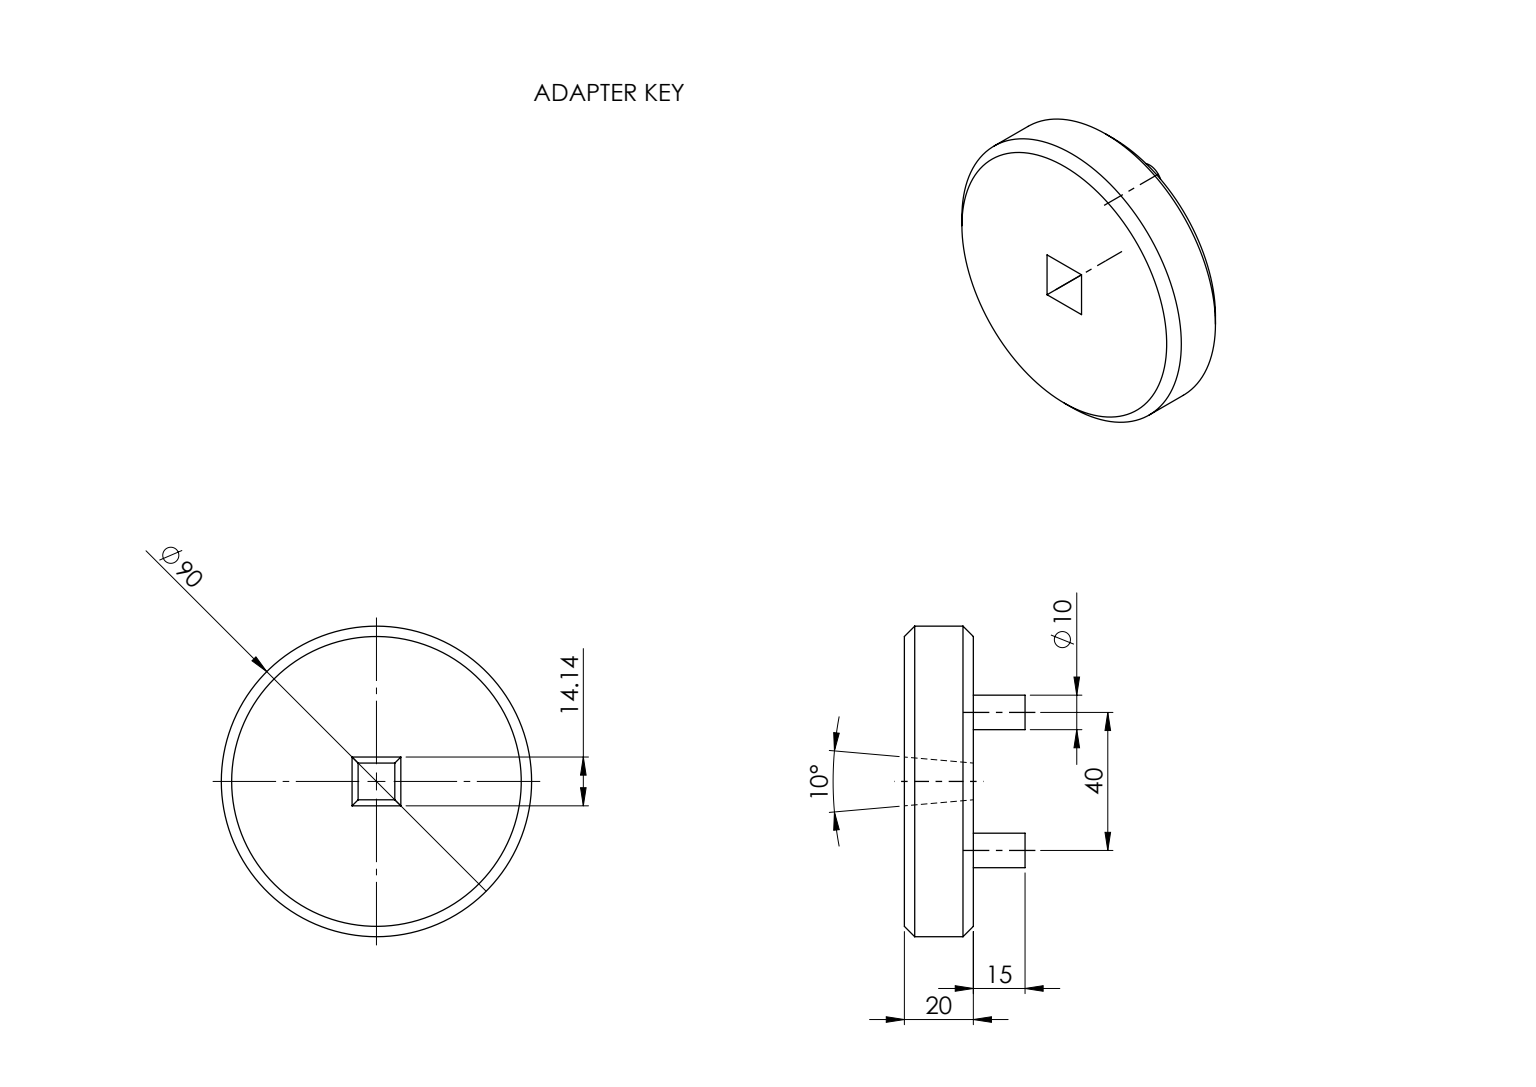
ISO-10303-21;
HEADER;
FILE_DESCRIPTION (('STEP AP203'),
    '1' );
FILE_NAME ('adapter key.step',
    '2026-09-28T05:57:06',
    ( '' ),
    ( '' ),
    'SwSTEP 2.0',
    'SolidWorks 2026',
    '' );
FILE_SCHEMA (( 'AUTOMOTIVE_DESIGN' ));
ENDSEC;

DATA;
#1=ORIENTED_EDGE ( 'NONE', *, *, #11918, .T. ) ;
#11=AXIS2_PLACEMENT_3D ( 'NONE', #22333, #25786, #11966 ) ;
#126=FACE_OUTER_BOUND ( 'NONE', #13645, .T. ) ;
#159=DIRECTION ( 'NONE',  ( -1.000000000000000000, 0.000000000000000000, 0.000000000000000000 ) ) ;
#483=ORIENTED_EDGE ( 'NONE', *, *, #39890, .F. ) ;
#526=CARTESIAN_POINT ( 'NONE',  ( 0.000000000000000000, 5.321294541346989426, -219.9999999999999716 ) ) ;
#674=CARTESIAN_POINT ( 'NONE',  ( 6.964452268037472749, 6.964452268037473637, -201.2186212422413689 ) ) ;
#785=DIRECTION ( 'NONE',  ( -0.000000000000000000, -0.000000000000000000, 1.000000000000000000 ) ) ;
#953=CARTESIAN_POINT ( 'NONE',  ( -5.000000000000002665, 20.00000000000000000, -235.0000000000000000 ) ) ;
#967=CARTESIAN_POINT ( 'NONE',  ( -2.275517850991317657E-15, -20.00000000000000000, -235.0000000000000000 ) ) ;
#1100=VECTOR ( 'NONE', #32490, 1000.000000000000000 ) ;
#1141=ORIENTED_EDGE ( 'NONE', *, *, #16442, .T. ) ;
#1157=CARTESIAN_POINT ( 'NONE',  ( -45.00000000000000711, 0.000000000000000000, -203.0000000000000000 ) ) ;
#1331=DIRECTION ( 'NONE',  ( 0.000000000000000000, 0.000000000000000000, -1.000000000000000000 ) ) ;
#1487=MANIFOLD_SOLID_BREP ( 'Cavity1', #17003 ) ;
#1498=PRODUCT ( 'adapter key', 'adapter key', '', ( #33542 ) ) ;
#1541=EDGE_LOOP ( 'NONE', ( #15994, #2474, #42330, #20143 ) ) ;
#1544=AXIS2_PLACEMENT_3D ( 'NONE', #42021, #38801, #12243 ) ;
#1593=ORIENTED_EDGE ( 'NONE', *, *, #39837, .F. ) ;
#1636=CARTESIAN_POINT ( 'NONE',  ( -45.00000000000000711, 0.000000000000000000, -217.0000000000000853 ) ) ;
#1647=CARTESIAN_POINT ( 'NONE',  ( 5.000000000000000000, -20.00000000000000000, -235.0000000000000000 ) ) ;
#1763=AXIS2_PLACEMENT_3D ( 'NONE', #7556, #33682, #13996 ) ;
#2026=ADVANCED_FACE ( 'NONE', ( #8164 ), #10577, .F. ) ;
#2078=CARTESIAN_POINT ( 'NONE',  ( 0.000000000000000000, 0.000000000000000000, -200.0000000000000000 ) ) ;
#2080=VECTOR ( 'NONE', #35351, 1000.000000000000000 ) ;
#2296=DIRECTION ( 'NONE',  ( 0.000000000000000000, 0.000000000000000000, -1.000000000000000000 ) ) ;
#2379=DIRECTION ( 'NONE',  ( 0.000000000000000000, 0.000000000000000000, -1.000000000000000000 ) ) ;
#2410=CARTESIAN_POINT ( 'NONE',  ( 0.000000000000000000, 0.000000000000000000, -200.0000000000000000 ) ) ;
#2474=ORIENTED_EDGE ( 'NONE', *, *, #18806, .T. ) ;
#2480=EDGE_CURVE ( 'NONE', #35035, #8964, #11432, .T. ) ;
#2552=CARTESIAN_POINT ( 'NONE',  ( 42.00000000000004974, 0.000000000000000000, -219.9999999999999716 ) ) ;
#2589=FACE_OUTER_BOUND ( 'NONE', #11013, .T. ) ;
#2598=DIRECTION ( 'NONE',  ( 0.08682659386424779191, -0.08682659386424779191, 0.9924325091389669673 ) ) ;
#2602=ORIENTED_EDGE ( 'NONE', *, *, #11918, .F. ) ;
#2615=CARTESIAN_POINT ( 'NONE',  ( -7.071067811865477282, 7.071067811865471064, -200.0000000000000000 ) ) ;
#2639=DIRECTION ( 'NONE',  ( 0.000000000000000000, 0.000000000000000000, -1.000000000000000000 ) ) ;
#2651=EDGE_LOOP ( 'NONE', ( #20661, #18080, #34460, #33121 ) ) ;
#2652=EDGE_LOOP ( 'NONE', ( #37130, #21052, #35179, #1 ) ) ;
#2679=ORIENTED_EDGE ( 'NONE', *, *, #40709, .F. ) ;
#2703=DIRECTION ( 'NONE',  ( 0.000000000000000000, 0.000000000000000000, -1.000000000000000000 ) ) ;
#2844=FACE_OUTER_BOUND ( 'NONE', #29189, .T. ) ;
#2864=ADVANCED_FACE ( 'NONE', ( #37885 ), #20831, .F. ) ;
#2943=AXIS2_PLACEMENT_3D ( 'NONE', #28917, #28711, #6033 ) ;
#3110=AXIS2_PLACEMENT_3D ( 'NONE', #25408, #5334, #8580 ) ;
#3136=VECTOR ( 'NONE', #7346, 1000.000000000000114 ) ;
#3175=CARTESIAN_POINT ( 'NONE',  ( -2.275517850991317657E-15, -20.00000000000000000, -219.9999999999999716 ) ) ;
#3290=DIRECTION ( 'NONE',  ( -0.000000000000000000, -0.000000000000000000, 1.000000000000000000 ) ) ;
#3542=VERTEX_POINT ( 'NONE', #1157 ) ;
#3598=DIRECTION ( 'NONE',  ( -0.7071067811865483499, 8.659560562354942719E-17, 0.7071067811865466846 ) ) ;
#3686=CARTESIAN_POINT ( 'NONE',  ( 5.000000000000000000, -20.00000000000000000, -219.9999999999999716 ) ) ;
#3707=ADVANCED_FACE ( 'NONE', ( #31585 ), #42117, .F. ) ;
#3843=DIRECTION ( 'NONE',  ( 0.000000000000000000, 0.000000000000000000, -1.000000000000000000 ) ) ;
#4412=FACE_OUTER_BOUND ( 'NONE', #14165, .T. ) ;
#4607=CARTESIAN_POINT ( 'NONE',  ( -5.321294541346989426, -5.321294541346989426, -219.9999999999999716 ) ) ;
#4626=DIRECTION ( 'NONE',  ( -1.000000000000000000, 0.000000000000000000, 0.000000000000000000 ) ) ;
#4650=CARTESIAN_POINT ( 'NONE',  ( 7.071067811865472841, 7.071067811865472841, -200.0000000000000000 ) ) ;
#4654=CARTESIAN_POINT ( 'NONE',  ( -7.071067811865477282, -7.071067811865472841, -200.0000000000000000 ) ) ;
#4922=DIRECTION ( 'NONE',  ( 0.000000000000000000, -0.9961946980917455452, -0.08715574274765837404 ) ) ;
#5010=AXIS2_PLACEMENT_3D ( 'NONE', #18603, #2639, #41891 ) ;
#5035=DIRECTION ( 'NONE',  ( -0.9961946980917455452, 0.000000000000000000, -0.08715574274765837404 ) ) ;
#5279=ORIENTED_EDGE ( 'NONE', *, *, #9308, .F. ) ;
#5319=CARTESIAN_POINT ( 'NONE',  ( 0.000000000000000000, 0.000000000000000000, -219.9999999999999716 ) ) ;
#5334=DIRECTION ( 'NONE',  ( 0.000000000000000000, 0.000000000000000000, -1.000000000000000000 ) ) ;
#5395=ORIENTED_EDGE ( 'NONE', *, *, #30592, .T. ) ;
#5451=PLANE ( 'NONE',  #28654 ) ;
#5465=ORIENTED_EDGE ( 'NONE', *, *, #12760, .F. ) ;
#5647=CARTESIAN_POINT ( 'NONE',  ( 0.000000000000000000, 20.00000000000000000, -235.0000000000000000 ) ) ;
#5755=ORIENTED_EDGE ( 'NONE', *, *, #38350, .F. ) ;
#5887=ORIENTED_EDGE ( 'NONE', *, *, #16876, .F. ) ;
#5935=AXIS2_PLACEMENT_3D ( 'NONE', #14018, #2703, #6942 ) ;
#5940=( NAMED_UNIT ( * ) PLANE_ANGLE_UNIT ( ) SI_UNIT ( $, .RADIAN. ) );
#6033=DIRECTION ( 'NONE',  ( -1.000000000000000000, 0.000000000000000000, 0.000000000000000000 ) ) ;
#6444=CARTESIAN_POINT ( 'NONE',  ( 0.000000000000000000, 0.000000000000000000, -219.9999999999999716 ) ) ;
#6566=AXIS2_PLACEMENT_3D ( 'NONE', #10357, #39929, #7353 ) ;
#6633=DIRECTION ( 'NONE',  ( 1.000000000000000000, -0.000000000000000000, -0.000000000000000000 ) ) ;
#6797=VECTOR ( 'NONE', #10559, 1000.000000000000000 ) ;
#6839=FACE_OUTER_BOUND ( 'NONE', #22128, .T. ) ;
#6843=CIRCLE ( 'NONE', #42657, 5.000000000000002665 ) ;
#6856=DIRECTION ( 'NONE',  ( -1.000000000000000000, 0.000000000000000000, -0.000000000000000000 ) ) ;
#6863=EDGE_CURVE ( 'NONE', #25211, #17989, #19820, .T. ) ;
#6942=DIRECTION ( 'NONE',  ( -1.000000000000000000, 0.000000000000000000, 0.000000000000000000 ) ) ;
#6947=CARTESIAN_POINT ( 'NONE',  ( -2.275517850991317657E-15, -20.00000000000000000, -235.0000000000000000 ) ) ;
#6976=EDGE_CURVE ( 'NONE', #21643, #18815, #29301, .T. ) ;
#6984=LINE ( 'NONE', #526, #42165 ) ;
#7000=AXIS2_PLACEMENT_3D ( 'NONE', #27316, #785, #27529 ) ;
#7012=DIRECTION ( 'NONE',  ( -1.000000000000000000, 0.000000000000000000, -0.000000000000000000 ) ) ;
#7136=FACE_BOUND ( 'NONE', #35464, .T. ) ;
#7294=CARTESIAN_POINT ( 'NONE',  ( 7.071067811865477282, -7.071067811865471064, -200.0000000000000000 ) ) ;
#7346=DIRECTION ( 'NONE',  ( 0.08682659386424779191, 0.08682659386424779191, 0.9924325091389669673 ) ) ;
#7353=DIRECTION ( 'NONE',  ( -1.000000000000000000, 0.000000000000000000, -0.000000000000000000 ) ) ;
#7454=EDGE_CURVE ( 'NONE', #27111, #16738, #32754, .T. ) ;
#7556=CARTESIAN_POINT ( 'NONE',  ( -2.275517850991317657E-15, -20.00000000000000000, -235.0000000000000000 ) ) ;
#7576=CIRCLE ( 'NONE', #11, 5.000000000000002665 ) ;
#7595=DIRECTION ( 'NONE',  ( 0.9961946980917455452, 0.000000000000000000, -0.08715574274765837404 ) ) ;
#7679=DIRECTION ( 'NONE',  ( 0.000000000000000000, 0.9961946980917455452, -0.08715574274765837404 ) ) ;
#7755=EDGE_CURVE ( 'NONE', #14989, #27111, #11989, .T. ) ;
#7817=FACE_OUTER_BOUND ( 'NONE', #27002, .T. ) ;
#8134=DIRECTION ( 'NONE',  ( 0.000000000000000000, 0.000000000000000000, 1.000000000000000000 ) ) ;
#8164=FACE_OUTER_BOUND ( 'NONE', #20948, .T. ) ;
#8171=DIRECTION ( 'NONE',  ( 1.000000000000000000, 0.000000000000000000, 0.000000000000000000 ) ) ;
#8303=PRODUCT_DEFINITION ( 'UNKNOWN', '', #24948, #36055 ) ;
#8326=LINE ( 'NONE', #21042, #9603 ) ;
#8516=ORIENTED_EDGE ( 'NONE', *, *, #38069, .F. ) ;
#8544=ORIENTED_EDGE ( 'NONE', *, *, #12979, .T. ) ;
#8580=DIRECTION ( 'NONE',  ( -1.000000000000000000, 0.000000000000000000, 0.000000000000000000 ) ) ;
#8659=ORIENTED_EDGE ( 'NONE', *, *, #39837, .T. ) ;
#8684=CIRCLE ( 'NONE', #26592, 45.00000000000000711 ) ;
#8737=ORIENTED_EDGE ( 'NONE', *, *, #22756, .T. ) ;
#8756=CARTESIAN_POINT ( 'NONE',  ( 0.000000000000000000, 0.000000000000000000, -217.0000000000000853 ) ) ;
#8860=ORIENTED_EDGE ( 'NONE', *, *, #30592, .F. ) ;
#8964=VERTEX_POINT ( 'NONE', #34365 ) ;
#9066=ADVANCED_FACE ( 'NONE', ( #7817 ), #30906, .F. ) ;
#9301=EDGE_CURVE ( 'NONE', #13682, #12005, #6843, .T. ) ;
#9308=EDGE_CURVE ( 'NONE', #32599, #21643, #15789, .T. ) ;
#9399=DIRECTION ( 'NONE',  ( 0.000000000000000000, 0.000000000000000000, 1.000000000000000000 ) ) ;
#9603=VECTOR ( 'NONE', #11321, 1000.000000000000000 ) ;
#9635=CYLINDRICAL_SURFACE ( 'NONE', #7000, 5.000000000000002665 ) ;
#9644=EDGE_LOOP ( 'NONE', ( #21891, #30300, #22496, #15785 ) ) ;
#10152=FACE_OUTER_BOUND ( 'NONE', #39088, .T. ) ;
#10209=ORIENTED_EDGE ( 'NONE', *, *, #38350, .T. ) ;
#10271=ORIENTED_EDGE ( 'NONE', *, *, #41214, .F. ) ;
#10357=CARTESIAN_POINT ( 'NONE',  ( 0.000000000000000000, 0.000000000000000000, -219.9999999999999716 ) ) ;
#10378=ADVANCED_FACE ( 'NONE', ( #34632, #27507 ), #13521, .F. ) ;
#10417=CARTESIAN_POINT ( 'NONE',  ( 7.071067811865472841, -7.071067811865472841, -200.0000000000000000 ) ) ;
#10540=CARTESIAN_POINT ( 'NONE',  ( 5.000000000000002665, 20.00000000000000000, -219.9999999999999716 ) ) ;
#10559=DIRECTION ( 'NONE',  ( -0.000000000000000000, -0.000000000000000000, 1.000000000000000000 ) ) ;
#10577=PLANE ( 'NONE',  #12775 ) ;
#10589=DIRECTION ( 'NONE',  ( -1.000000000000000000, 0.000000000000000000, 0.000000000000000000 ) ) ;
#10590=ADVANCED_FACE ( 'NONE', ( #4412 ), #22716, .T. ) ;
#10848=AXIS2_PLACEMENT_3D ( 'NONE', #6947, #1331, #10589 ) ;
#10918=DIRECTION ( 'NONE',  ( -0.000000000000000000, -1.000000000000000000, -0.000000000000000000 ) ) ;
#11013=EDGE_LOOP ( 'NONE', ( #11087, #37618, #18353, #1593 ) ) ;
#11087=ORIENTED_EDGE ( 'NONE', *, *, #23326, .F. ) ;
#11112=DIRECTION ( 'NONE',  ( 0.000000000000000000, 0.000000000000000000, 1.000000000000000000 ) ) ;
#11133=LINE ( 'NONE', #18253, #42479 ) ;
#11321=DIRECTION ( 'NONE',  ( -1.000000000000000000, 0.000000000000000000, 0.000000000000000000 ) ) ;
#11331=ORIENTED_EDGE ( 'NONE', *, *, #20682, .F. ) ;
#11377=CIRCLE ( 'NONE', #1763, 5.000000000000002665 ) ;
#11382=CARTESIAN_POINT ( 'NONE',  ( -2.275517850991317657E-15, -20.00000000000000000, -235.0000000000000000 ) ) ;
#11432=CIRCLE ( 'NONE', #12117, 5.000000000000002665 ) ;
#11492=DIRECTION ( 'NONE',  ( -0.08682659386424779191, -0.08682659386424779191, 0.9924325091389669673 ) ) ;
#11559=AXIS2_PLACEMENT_3D ( 'NONE', #40001, #42386, #22553 ) ;
#11596=ORIENTED_EDGE ( 'NONE', *, *, #2480, .F. ) ;
#11632=CARTESIAN_POINT ( 'NONE',  ( -45.00000000000000711, 0.000000000000000000, -200.0000000000000000 ) ) ;
#11721=VECTOR ( 'NONE', #18934, 1000.000000000000114 ) ;
#11857=APPLICATION_CONTEXT ( 'configuration controlled 3d designs of mechanical parts and assemblies' ) ;
#11870=EDGE_CURVE ( 'NONE', #17989, #25211, #11377, .T. ) ;
#11918=EDGE_CURVE ( 'NONE', #28029, #16738, #39924, .T. ) ;
#11966=DIRECTION ( 'NONE',  ( -1.000000000000000000, 0.000000000000000000, 0.000000000000000000 ) ) ;
#11989=LINE ( 'NONE', #38534, #22609 ) ;
#11992=FACE_OUTER_BOUND ( 'NONE', #35700, .T. ) ;
#12005=VERTEX_POINT ( 'NONE', #15500 ) ;
#12066=CARTESIAN_POINT ( 'NONE',  ( 45.00000000000000711, 5.510910596163090344E-15, -203.0000000000000000 ) ) ;
#12076=ORIENTED_EDGE ( 'NONE', *, *, #9301, .F. ) ;
#12117=AXIS2_PLACEMENT_3D ( 'NONE', #3175, #13911, #159 ) ;
#12133=EDGE_LOOP ( 'NONE', ( #33495, #8860, #16467, #13801 ) ) ;
#12243=DIRECTION ( 'NONE',  ( -1.000000000000000000, 0.000000000000000000, 0.000000000000000000 ) ) ;
#12301=VECTOR ( 'NONE', #30444, 1000.000000000000000 ) ;
#12357=CARTESIAN_POINT ( 'NONE',  ( 0.000000000000000000, 0.000000000000000000, -200.0000000000000000 ) ) ;
#12505=CARTESIAN_POINT ( 'NONE',  ( 0.000000000000000000, 0.000000000000000000, -219.9999999999999716 ) ) ;
#12537=DIRECTION ( 'NONE',  ( -1.000000000000000000, 0.000000000000000000, -0.000000000000000000 ) ) ;
#12651=VERTEX_POINT ( 'NONE', #7294 ) ;
#12747=AXIS2_PLACEMENT_3D ( 'NONE', #41976, #9399, #35532 ) ;
#12760=EDGE_CURVE ( 'NONE', #23937, #42482, #35502, .T. ) ;
#12775=AXIS2_PLACEMENT_3D ( 'NONE', #24574, #4922, #37722 ) ;
#12979=EDGE_CURVE ( 'NONE', #16950, #13797, #16502, .T. ) ;
#13267=DIRECTION ( 'NONE',  ( -1.000000000000000000, -0.000000000000000000, -0.000000000000000000 ) ) ;
#13298=DIRECTION ( 'NONE',  ( -0.000000000000000000, -0.000000000000000000, -1.000000000000000000 ) ) ;
#13521=PLANE ( 'NONE',  #24803 ) ;
#13645=EDGE_LOOP ( 'NONE', ( #17252, #15517 ) ) ;
#13656=FACE_OUTER_BOUND ( 'NONE', #1541, .T. ) ;
#13682=VERTEX_POINT ( 'NONE', #953 ) ;
#13797=VERTEX_POINT ( 'NONE', #4607 ) ;
#13801=ORIENTED_EDGE ( 'NONE', *, *, #7755, .T. ) ;
#13832=( GEOMETRIC_REPRESENTATION_CONTEXT ( 3 ) GLOBAL_UNCERTAINTY_ASSIGNED_CONTEXT ( ( #33340 ) ) GLOBAL_UNIT_ASSIGNED_CONTEXT ( ( #31640, #5940, #25165 ) ) REPRESENTATION_CONTEXT ( 'NONE', 'WORKASPACE' ) );
#13911=DIRECTION ( 'NONE',  ( 0.000000000000000000, 0.000000000000000000, -1.000000000000000000 ) ) ;
#13930=VECTOR ( 'NONE', #2379, 1000.000000000000000 ) ;
#13996=DIRECTION ( 'NONE',  ( -1.000000000000000000, 0.000000000000000000, 0.000000000000000000 ) ) ;
#14018=CARTESIAN_POINT ( 'NONE',  ( 0.000000000000000000, 20.00000000000000000, -219.9999999999999716 ) ) ;
#14158=AXIS2_PLACEMENT_3D ( 'NONE', #31807, #5035, #28979 ) ;
#14165=EDGE_LOOP ( 'NONE', ( #30572, #5279, #8659, #38093 ) ) ;
#14623=ADVANCED_FACE ( 'NONE', ( #38005 ), #35268, .T. ) ;
#14777=DIRECTION ( 'NONE',  ( -0.000000000000000000, -0.000000000000000000, 1.000000000000000000 ) ) ;
#14868=DIRECTION ( 'NONE',  ( 0.000000000000000000, 0.000000000000000000, -1.000000000000000000 ) ) ;
#14989=VERTEX_POINT ( 'NONE', #39478 ) ;
#15381=ADVANCED_FACE ( 'NONE', ( #42426 ), #9635, .T. ) ;
#15500=CARTESIAN_POINT ( 'NONE',  ( 5.000000000000002665, 20.00000000000000000, -235.0000000000000000 ) ) ;
#15517=ORIENTED_EDGE ( 'NONE', *, *, #11870, .T. ) ;
#15528=DIRECTION ( 'NONE',  ( 0.000000000000000000, 0.000000000000000000, 1.000000000000000000 ) ) ;
#15785=ORIENTED_EDGE ( 'NONE', *, *, #2480, .T. ) ;
#15789=CIRCLE ( 'NONE', #33719, 42.00000000000001421 ) ;
#15836=CIRCLE ( 'NONE', #39980, 5.000000000000002665 ) ;
#15858=ORIENTED_EDGE ( 'NONE', *, *, #35195, .T. ) ;
#15994=ORIENTED_EDGE ( 'NONE', *, *, #29097, .T. ) ;
#16130=ORIENTED_EDGE ( 'NONE', *, *, #31655, .F. ) ;
#16145=EDGE_CURVE ( 'NONE', #14989, #28029, #6984, .T. ) ;
#16200=ORIENTED_EDGE ( 'NONE', *, *, #18037, .T. ) ;
#16205=CARTESIAN_POINT ( 'NONE',  ( -2.275517850991317657E-15, -20.00000000000000000, -235.0000000000000000 ) ) ;
#16309=ORIENTED_EDGE ( 'NONE', *, *, #12760, .T. ) ;
#16354=VECTOR ( 'NONE', #11492, 1000.000000000000114 ) ;
#16442=EDGE_CURVE ( 'NONE', #16950, #12651, #39986, .T. ) ;
#16467=ORIENTED_EDGE ( 'NONE', *, *, #22649, .T. ) ;
#16502=LINE ( 'NONE', #32522, #26548 ) ;
#16738=VERTEX_POINT ( 'NONE', #32984 ) ;
#16876=EDGE_CURVE ( 'NONE', #42482, #23937, #26361, .T. ) ;
#16950=VERTEX_POINT ( 'NONE', #21243 ) ;
#16977=DIRECTION ( 'NONE',  ( -1.000000000000000000, 0.000000000000000000, 0.000000000000000000 ) ) ;
#17003=CLOSED_SHELL ( 'NONE', ( #18808, #14623, #29395, #30885, #30210, #10378, #24136, #20403, #42288, #22994, #15381, #23992, #22502, #10590, #3707, #2864, #9066, #2026 ) ) ;
#17162=ORIENTED_EDGE ( 'NONE', *, *, #20682, .T. ) ;
#17252=ORIENTED_EDGE ( 'NONE', *, *, #6863, .T. ) ;
#17551=CARTESIAN_POINT ( 'NONE',  ( 0.000000000000000000, 0.000000000000000000, -203.0000000000000000 ) ) ;
#17817=LINE ( 'NONE', #31440, #32266 ) ;
#17898=APPLICATION_CONTEXT ( 'configuration controlled 3d designs of mechanical parts and assemblies' ) ;
#17989=VERTEX_POINT ( 'NONE', #31791 ) ;
#18025=DIRECTION ( 'NONE',  ( -1.000000000000000000, 0.000000000000000000, 0.000000000000000000 ) ) ;
#18037=EDGE_CURVE ( 'NONE', #8964, #35035, #27055, .T. ) ;
#18080=ORIENTED_EDGE ( 'NONE', *, *, #22649, .F. ) ;
#18187=LINE ( 'NONE', #41048, #16354 ) ;
#18253=CARTESIAN_POINT ( 'NONE',  ( -5.321294541346989426, 0.000000000000000000, -219.9999999999999716 ) ) ;
#18353=ORIENTED_EDGE ( 'NONE', *, *, #29097, .F. ) ;
#18496=ORIENTED_EDGE ( 'NONE', *, *, #11870, .F. ) ;
#18509=EDGE_CURVE ( 'NONE', #3542, #38155, #24192, .T. ) ;
#18603=CARTESIAN_POINT ( 'NONE',  ( -2.275517850991317657E-15, -20.00000000000000000, -219.9999999999999716 ) ) ;
#18667=DIRECTION ( 'NONE',  ( -1.000000000000000000, 0.000000000000000000, 0.000000000000000000 ) ) ;
#18795=DIRECTION ( 'NONE',  ( -1.000000000000000000, 0.000000000000000000, 0.000000000000000000 ) ) ;
#18806=EDGE_CURVE ( 'NONE', #18815, #38638, #22005, .T. ) ;
#18808=ADVANCED_FACE ( 'NONE', ( #2589 ), #31888, .T. ) ;
#18815=VERTEX_POINT ( 'NONE', #12066 ) ;
#18886=EDGE_LOOP ( 'NONE', ( #5465, #36501, #39209, #29608 ) ) ;
#18934=DIRECTION ( 'NONE',  ( -0.7071067811865459074, 0.000000000000000000, -0.7071067811865491270 ) ) ;
#19139=CARTESIAN_POINT ( 'NONE',  ( 0.000000000000000000, 20.00000000000000000, -219.9999999999999716 ) ) ;
#19299=CYLINDRICAL_SURFACE ( 'NONE', #11559, 45.00000000000000711 ) ;
#19340=AXIS2_PLACEMENT_3D ( 'NONE', #11382, #24580, #8171 ) ;
#19343=DIRECTION ( 'NONE',  ( 0.000000000000000000, 0.000000000000000000, -1.000000000000000000 ) ) ;
#19407=AXIS2_PLACEMENT_3D ( 'NONE', #12505, #15528, #38427 ) ;
#19554=LINE ( 'NONE', #38996, #2080 ) ;
#19713=CARTESIAN_POINT ( 'NONE',  ( 45.00000000000000711, 5.510910596163090344E-15, -217.0000000000000853 ) ) ;
#19820=CIRCLE ( 'NONE', #10848, 5.000000000000002665 ) ;
#19946=VECTOR ( 'NONE', #3598, 1000.000000000000000 ) ;
#19992=CYLINDRICAL_SURFACE ( 'NONE', #28417, 5.000000000000002665 ) ;
#20143=ORIENTED_EDGE ( 'NONE', *, *, #18509, .F. ) ;
#20241=ORIENTED_EDGE ( 'NONE', *, *, #20405, .F. ) ;
#20300=EDGE_CURVE ( 'NONE', #38638, #38155, #8684, .T. ) ;
#20403=ADVANCED_FACE ( 'NONE', ( #31645 ), #35518, .T. ) ;
#20405=EDGE_CURVE ( 'NONE', #25211, #35035, #31220, .T. ) ;
#20412=VERTEX_POINT ( 'NONE', #27973 ) ;
#20419=EDGE_CURVE ( 'NONE', #37668, #27111, #41100, .T. ) ;
#20520=VECTOR ( 'NONE', #6633, 1000.000000000000000 ) ;
#20580=DIRECTION ( 'NONE',  ( 0.000000000000000000, 0.000000000000000000, -1.000000000000000000 ) ) ;
#20661=ORIENTED_EDGE ( 'NONE', *, *, #16145, .F. ) ;
#20682=EDGE_CURVE ( 'NONE', #21356, #20412, #24546, .T. ) ;
#20831=PLANE ( 'NONE',  #38306 ) ;
#20887=DIRECTION ( 'NONE',  ( -0.000000000000000000, -0.000000000000000000, 1.000000000000000000 ) ) ;
#20948=EDGE_LOOP ( 'NONE', ( #5755, #38517, #8544, #5395 ) ) ;
#21042=CARTESIAN_POINT ( 'NONE',  ( 7.071067811865472841, -7.071067811865472841, -200.0000000000000000 ) ) ;
#21052=ORIENTED_EDGE ( 'NONE', *, *, #7755, .F. ) ;
#21243=CARTESIAN_POINT ( 'NONE',  ( 5.321294541346989426, -5.321294541346989426, -219.9999999999999716 ) ) ;
#21356=VERTEX_POINT ( 'NONE', #10540 ) ;
#21384=DIRECTION ( 'NONE',  ( 0.7071067811865459074, 8.659560562354911904E-17, -0.7071067811865491270 ) ) ;
#21643=VERTEX_POINT ( 'NONE', #37953 ) ;
#21842=CARTESIAN_POINT ( 'NONE',  ( 0.000000000000000000, 20.00000000000000000, -235.0000000000000000 ) ) ;
#21891=ORIENTED_EDGE ( 'NONE', *, *, #35192, .F. ) ;
#22005=LINE ( 'NONE', #32583, #13930 ) ;
#22096=DIRECTION ( 'NONE',  ( -0.000000000000000000, -0.000000000000000000, 1.000000000000000000 ) ) ;
#22128=EDGE_LOOP ( 'NONE', ( #12076, #38318, #23767, #483 ) ) ;
#22333=CARTESIAN_POINT ( 'NONE',  ( 0.000000000000000000, 20.00000000000000000, -235.0000000000000000 ) ) ;
#22438=AXIS2_PLACEMENT_3D ( 'NONE', #12357, #22096, #23313 ) ;
#22473=AXIS2_PLACEMENT_3D ( 'NONE', #2078, #2296, #18025 ) ;
#22496=ORIENTED_EDGE ( 'NONE', *, *, #20405, .T. ) ;
#22502=ADVANCED_FACE ( 'NONE', ( #11992 ), #41769, .T. ) ;
#22550=CARTESIAN_POINT ( 'NONE',  ( -7.071067811865472841, -7.071067811865472841, -200.0000000000000000 ) ) ;
#22553=DIRECTION ( 'NONE',  ( -1.000000000000000000, 0.000000000000000000, 0.000000000000000000 ) ) ;
#22609=VECTOR ( 'NONE', #38116, 1000.000000000000114 ) ;
#22649=EDGE_CURVE ( 'NONE', #13797, #14989, #11133, .T. ) ;
#22716=CONICAL_SURFACE ( 'NONE', #40617, 45.00000000000000711, 0.7853981633974459475 ) ;
#22756=EDGE_CURVE ( 'NONE', #38155, #38638, #31482, .T. ) ;
#22911=FACE_BOUND ( 'NONE', #28242, .T. ) ;
#22994=ADVANCED_FACE ( 'NONE', ( #126 ), #33770, .T. ) ;
#23138=DIRECTION ( 'NONE',  ( 1.000000000000000000, 0.000000000000000000, 0.000000000000000000 ) ) ;
#23313=DIRECTION ( 'NONE',  ( -1.000000000000000000, 0.000000000000000000, 0.000000000000000000 ) ) ;
#23326=EDGE_CURVE ( 'NONE', #21643, #32599, #29309, .T. ) ;
#23333=FACE_BOUND ( 'NONE', #2651, .T. ) ;
#23352=VECTOR ( 'NONE', #29633, 1000.000000000000000 ) ;
#23615=VECTOR ( 'NONE', #14868, 1000.000000000000000 ) ;
#23680=DIRECTION ( 'NONE',  ( -1.000000000000000000, 0.000000000000000000, 0.000000000000000000 ) ) ;
#23745=LINE ( 'NONE', #36898, #12301 ) ;
#23767=ORIENTED_EDGE ( 'NONE', *, *, #41214, .T. ) ;
#23885=PRODUCT_DEFINITION_SHAPE ( 'NONE', 'NONE',  #8303 ) ;
#23894=AXIS2_PLACEMENT_3D ( 'NONE', #5319, #8134, #34686 ) ;
#23937=VERTEX_POINT ( 'NONE', #41889 ) ;
#23992=ADVANCED_FACE ( 'NONE', ( #2844 ), #5451, .T. ) ;
#24093=ORIENTED_EDGE ( 'NONE', *, *, #18806, .F. ) ;
#24136=ADVANCED_FACE ( 'NONE', ( #10152, #7136, #22911, #23333 ), #36907, .T. ) ;
#24189=ORIENTED_EDGE ( 'NONE', *, *, #35192, .T. ) ;
#24192=LINE ( 'NONE', #11632, #23615 ) ;
#24335=DIRECTION ( 'NONE',  ( -0.000000000000000000, 1.000000000000000000, -0.000000000000000000 ) ) ;
#24426=ORIENTED_EDGE ( 'NONE', *, *, #9308, .T. ) ;
#24546=CIRCLE ( 'NONE', #5935, 5.000000000000002665 ) ;
#24574=CARTESIAN_POINT ( 'NONE',  ( 7.071067811865472841, -7.071067811865472841, -200.0000000000000000 ) ) ;
#24580=DIRECTION ( 'NONE',  ( -0.000000000000000000, -0.000000000000000000, 1.000000000000000000 ) ) ;
#24743=CARTESIAN_POINT ( 'NONE',  ( 0.000000000000000000, 0.000000000000000000, 0.000000000000000000 ) ) ;
#24803=AXIS2_PLACEMENT_3D ( 'NONE', #37205, #37429, #6856 ) ;
#24948=PRODUCT_DEFINITION_FORMATION_WITH_SPECIFIED_SOURCE ( 'ANY', '', #1498, .NOT_KNOWN. ) ;
#25165=( NAMED_UNIT ( * ) SI_UNIT ( $, .STERADIAN. ) SOLID_ANGLE_UNIT ( ) );
#25211=VERTEX_POINT ( 'NONE', #41304 ) ;
#25352=EDGE_LOOP ( 'NONE', ( #24426, #34709 ) ) ;
#25408=CARTESIAN_POINT ( 'NONE',  ( 0.000000000000000000, 0.000000000000000000, -219.9999999999999716 ) ) ;
#25786=DIRECTION ( 'NONE',  ( 0.000000000000000000, 0.000000000000000000, -1.000000000000000000 ) ) ;
#25842=ORIENTED_EDGE ( 'NONE', *, *, #7454, .T. ) ;
#25864=AXIS2_PLACEMENT_3D ( 'NONE', #967, #20580, #7012 ) ;
#26162=ORIENTED_EDGE ( 'NONE', *, *, #16876, .T. ) ;
#26361=CIRCLE ( 'NONE', #27026, 42.00000000000004974 ) ;
#26548=VECTOR ( 'NONE', #13267, 1000.000000000000000 ) ;
#26592=AXIS2_PLACEMENT_3D ( 'NONE', #8756, #37894, #18667 ) ;
#26691=DIRECTION ( 'NONE',  ( -0.000000000000000000, -0.000000000000000000, 1.000000000000000000 ) ) ;
#26971=LINE ( 'NONE', #40129, #6797 ) ;
#27002=EDGE_LOOP ( 'NONE', ( #16130, #2602, #15858, #1141 ) ) ;
#27026=AXIS2_PLACEMENT_3D ( 'NONE', #6444, #3843, #16977 ) ;
#27055=CIRCLE ( 'NONE', #5010, 5.000000000000002665 ) ;
#27111=VERTEX_POINT ( 'NONE', #2615 ) ;
#27316=CARTESIAN_POINT ( 'NONE',  ( 0.000000000000000000, 20.00000000000000000, -235.0000000000000000 ) ) ;
#27452=DIRECTION ( 'NONE',  ( -0.08715574274765837404, 0.000000000000000000, -0.9961946980917455452 ) ) ;
#27507=FACE_OUTER_BOUND ( 'NONE', #25352, .T. ) ;
#27529=DIRECTION ( 'NONE',  ( 1.000000000000000000, 0.000000000000000000, 0.000000000000000000 ) ) ;
#27540=EDGE_LOOP ( 'NONE', ( #24093, #28832, #36743, #8737 ) ) ;
#27591=CARTESIAN_POINT ( 'NONE',  ( -5.000000000000002665, 20.00000000000000000, -235.0000000000000000 ) ) ;
#27603=VECTOR ( 'NONE', #20887, 1000.000000000000000 ) ;
#27796=ORIENTED_EDGE ( 'NONE', *, *, #22756, .F. ) ;
#27926=CARTESIAN_POINT ( 'NONE',  ( -42.00000000000001421, 0.000000000000000000, -200.0000000000000000 ) ) ;
#27973=CARTESIAN_POINT ( 'NONE',  ( -5.000000000000002665, 20.00000000000000000, -219.9999999999999716 ) ) ;
#28029=VERTEX_POINT ( 'NONE', #30568 ) ;
#28194=EDGE_LOOP ( 'NONE', ( #18496, #24189, #16200, #20241 ) ) ;
#28242=EDGE_LOOP ( 'NONE', ( #11596, #39839 ) ) ;
#28278=ORIENTED_EDGE ( 'NONE', *, *, #20419, .T. ) ;
#28311=DIRECTION ( 'NONE',  ( -0.000000000000000000, -0.000000000000000000, 1.000000000000000000 ) ) ;
#28417=AXIS2_PLACEMENT_3D ( 'NONE', #33183, #26691, #39844 ) ;
#28464=ORIENTED_EDGE ( 'NONE', *, *, #42273, .F. ) ;
#28654=AXIS2_PLACEMENT_3D ( 'NONE', #21842, #29174, #12537 ) ;
#28711=DIRECTION ( 'NONE',  ( -0.000000000000000000, -0.000000000000000000, -1.000000000000000000 ) ) ;
#28832=ORIENTED_EDGE ( 'NONE', *, *, #31491, .T. ) ;
#28917=CARTESIAN_POINT ( 'NONE',  ( 0.000000000000000000, 0.000000000000000000, -203.0000000000000000 ) ) ;
#28979=DIRECTION ( 'NONE',  ( 0.08715574274765837404, 0.000000000000000000, -0.9961946980917455452 ) ) ;
#29097=EDGE_CURVE ( 'NONE', #3542, #18815, #31873, .T. ) ;
#29174=DIRECTION ( 'NONE',  ( 0.000000000000000000, 0.000000000000000000, -1.000000000000000000 ) ) ;
#29189=EDGE_LOOP ( 'NONE', ( #29505, #32836 ) ) ;
#29301=LINE ( 'NONE', #42236, #30202 ) ;
#29309=CIRCLE ( 'NONE', #22438, 42.00000000000001421 ) ;
#29395=ADVANCED_FACE ( 'NONE', ( #6839 ), #19992, .T. ) ;
#29436=ADVANCED_BREP_SHAPE_REPRESENTATION ( '', ( #1487, #39998 ), #13832 ) ;
#29495=LINE ( 'NONE', #33167, #19946 ) ;
#29505=ORIENTED_EDGE ( 'NONE', *, *, #40709, .T. ) ;
#29512=AXIS2_PLACEMENT_3D ( 'NONE', #36409, #13298, #23680 ) ;
#29608=ORIENTED_EDGE ( 'NONE', *, *, #34141, .F. ) ;
#29633=DIRECTION ( 'NONE',  ( 0.7071067811865483499, 0.000000000000000000, 0.7071067811865466846 ) ) ;
#29852=LINE ( 'NONE', #32875, #23352 ) ;
#30202=VECTOR ( 'NONE', #21384, 1000.000000000000114 ) ;
#30210=ADVANCED_FACE ( 'NONE', ( #13656 ), #19299, .T. ) ;
#30300=ORIENTED_EDGE ( 'NONE', *, *, #6863, .F. ) ;
#30303=AXIS2_PLACEMENT_3D ( 'NONE', #37587, #7595, #27452 ) ;
#30444=DIRECTION ( 'NONE',  ( -0.000000000000000000, -1.000000000000000000, -0.000000000000000000 ) ) ;
#30568=CARTESIAN_POINT ( 'NONE',  ( 5.321294541346989426, 5.321294541346989426, -219.9999999999999716 ) ) ;
#30572=ORIENTED_EDGE ( 'NONE', *, *, #6976, .F. ) ;
#30592=EDGE_CURVE ( 'NONE', #13797, #37668, #18187, .T. ) ;
#30752=DIRECTION ( 'NONE',  ( -0.000000000000000000, -0.000000000000000000, -1.000000000000000000 ) ) ;
#30879=CIRCLE ( 'NONE', #29512, 45.00000000000000711 ) ;
#30885=ADVANCED_FACE ( 'NONE', ( #35677 ), #39105, .T. ) ;
#30906=PLANE ( 'NONE',  #30303 ) ;
#31165=VECTOR ( 'NONE', #2598, 1000.000000000000114 ) ;
#31220=LINE ( 'NONE', #1647, #39677 ) ;
#31440=CARTESIAN_POINT ( 'NONE',  ( 7.071067811865472841, -7.071067811865472841, -200.0000000000000000 ) ) ;
#31477=LINE ( 'NONE', #35774, #11721 ) ;
#31480=LINE ( 'NONE', #27591, #27603 ) ;
#31482=CIRCLE ( 'NONE', #12747, 45.00000000000000711 ) ;
#31491=EDGE_CURVE ( 'NONE', #18815, #3542, #30879, .T. ) ;
#31557=DIRECTION ( 'NONE',  ( -1.000000000000000000, 0.000000000000000000, 0.000000000000000000 ) ) ;
#31585=FACE_OUTER_BOUND ( 'NONE', #12133, .T. ) ;
#31640=( LENGTH_UNIT ( ) NAMED_UNIT ( * ) SI_UNIT ( .MILLI., .METRE. ) );
#31645=FACE_OUTER_BOUND ( 'NONE', #27540, .T. ) ;
#31655=EDGE_CURVE ( 'NONE', #16738, #12651, #17817, .T. ) ;
#31791=CARTESIAN_POINT ( 'NONE',  ( -5.000000000000005329, -20.00000000000000000, -235.0000000000000000 ) ) ;
#31807=CARTESIAN_POINT ( 'NONE',  ( -7.071067811865472841, -7.071067811865472841, -200.0000000000000000 ) ) ;
#31873=CIRCLE ( 'NONE', #1544, 45.00000000000000711 ) ;
#31888=CONICAL_SURFACE ( 'NONE', #2943, 45.00000000000000711, 0.7853981633974459475 ) ;
#31968=ORIENTED_EDGE ( 'NONE', *, *, #39890, .T. ) ;
#31984=DIRECTION ( 'NONE',  ( 0.000000000000000000, 0.000000000000000000, -1.000000000000000000 ) ) ;
#32175=SHAPE_DEFINITION_REPRESENTATION ( #23885, #36293 ) ;
#32266=VECTOR ( 'NONE', #10918, 1000.000000000000000 ) ;
#32479=DIRECTION ( 'NONE',  ( 1.000000000000000000, -0.000000000000000000, -0.000000000000000000 ) ) ;
#32490=DIRECTION ( 'NONE',  ( 0.000000000000000000, 1.000000000000000000, 0.000000000000000000 ) ) ;
#32522=CARTESIAN_POINT ( 'NONE',  ( 0.000000000000000000, -5.321294541346989426, -219.9999999999999716 ) ) ;
#32583=CARTESIAN_POINT ( 'NONE',  ( 45.00000000000000711, 5.510910596163090344E-15, -200.0000000000000000 ) ) ;
#32599=VERTEX_POINT ( 'NONE', #27926 ) ;
#32754=LINE ( 'NONE', #39432, #20520 ) ;
#32836=ORIENTED_EDGE ( 'NONE', *, *, #9301, .T. ) ;
#32875=CARTESIAN_POINT ( 'NONE',  ( 42.00000000000004974, 0.000000000000000000, -219.9999999999999716 ) ) ;
#32984=CARTESIAN_POINT ( 'NONE',  ( 7.071067811865472841, 7.071067811865472841, -200.0000000000000000 ) ) ;
#33121=ORIENTED_EDGE ( 'NONE', *, *, #35195, .F. ) ;
#33167=CARTESIAN_POINT ( 'NONE',  ( -42.00000000000004974, 5.143516556418889633E-15, -219.9999999999999716 ) ) ;
#33183=CARTESIAN_POINT ( 'NONE',  ( 0.000000000000000000, 20.00000000000000000, -235.0000000000000000 ) ) ;
#33340=UNCERTAINTY_MEASURE_WITH_UNIT (LENGTH_MEASURE( 1.000000000000000082E-05 ), #31640, 'distance_accuracy_value', 'NONE');
#33495=ORIENTED_EDGE ( 'NONE', *, *, #20419, .F. ) ;
#33542=MECHANICAL_CONTEXT ( 'NONE', #11857, 'mechanical' ) ;
#33682=DIRECTION ( 'NONE',  ( 0.000000000000000000, 0.000000000000000000, -1.000000000000000000 ) ) ;
#33699=ORIENTED_EDGE ( 'NONE', *, *, #34141, .T. ) ;
#33719=AXIS2_PLACEMENT_3D ( 'NONE', #2410, #28311, #18795 ) ;
#33770=PLANE ( 'NONE',  #25864 ) ;
#34016=DIRECTION ( 'NONE',  ( 0.000000000000000000, -0.08715574274765837404, -0.9961946980917455452 ) ) ;
#34141=EDGE_CURVE ( 'NONE', #42482, #38638, #29852, .T. ) ;
#34291=FACE_OUTER_BOUND ( 'NONE', #9644, .T. ) ;
#34365=CARTESIAN_POINT ( 'NONE',  ( -5.000000000000005329, -20.00000000000000000, -219.9999999999999716 ) ) ;
#34460=ORIENTED_EDGE ( 'NONE', *, *, #12979, .F. ) ;
#34632=FACE_BOUND ( 'NONE', #35194, .T. ) ;
#34686=DIRECTION ( 'NONE',  ( 1.000000000000000000, 0.000000000000000000, 0.000000000000000000 ) ) ;
#34709=ORIENTED_EDGE ( 'NONE', *, *, #23326, .T. ) ;
#35035=VERTEX_POINT ( 'NONE', #3686 ) ;
#35179=ORIENTED_EDGE ( 'NONE', *, *, #16145, .T. ) ;
#35192=EDGE_CURVE ( 'NONE', #17989, #8964, #26971, .T. ) ;
#35194=EDGE_LOOP ( 'NONE', ( #28278, #25842, #40340, #10209 ) ) ;
#35195=EDGE_CURVE ( 'NONE', #28029, #16950, #23745, .T. ) ;
#35268=CONICAL_SURFACE ( 'NONE', #19407, 42.00000000000004974, 0.7853981633974495002 ) ;
#35351=DIRECTION ( 'NONE',  ( -0.000000000000000000, -0.000000000000000000, 1.000000000000000000 ) ) ;
#35464=EDGE_LOOP ( 'NONE', ( #11331, #10271 ) ) ;
#35502=CIRCLE ( 'NONE', #3110, 42.00000000000004974 ) ;
#35518=CYLINDRICAL_SURFACE ( 'NONE', #22473, 45.00000000000000711 ) ;
#35532=DIRECTION ( 'NONE',  ( -1.000000000000000000, 0.000000000000000000, 0.000000000000000000 ) ) ;
#35677=FACE_OUTER_BOUND ( 'NONE', #28194, .T. ) ;
#35700=EDGE_LOOP ( 'NONE', ( #8516, #5887, #33699, #27796 ) ) ;
#35774=CARTESIAN_POINT ( 'NONE',  ( -45.00000000000000711, 0.000000000000000000, -203.0000000000000000 ) ) ;
#36055=DESIGN_CONTEXT ( 'detailed design', #17898, 'design' ) ;
#36293=SHAPE_REPRESENTATION ( 'adapter key', ( #39998 ), #13832 ) ;
#36409=CARTESIAN_POINT ( 'NONE',  ( 0.000000000000000000, 0.000000000000000000, -203.0000000000000000 ) ) ;
#36501=ORIENTED_EDGE ( 'NONE', *, *, #38069, .T. ) ;
#36743=ORIENTED_EDGE ( 'NONE', *, *, #18509, .T. ) ;
#36898=CARTESIAN_POINT ( 'NONE',  ( 5.321294541346989426, 0.000000000000000000, -219.9999999999999716 ) ) ;
#36907=PLANE ( 'NONE',  #6566 ) ;
#37129=EDGE_LOOP ( 'NONE', ( #28464, #2679, #31968, #17162 ) ) ;
#37130=ORIENTED_EDGE ( 'NONE', *, *, #7454, .F. ) ;
#37205=CARTESIAN_POINT ( 'NONE',  ( 0.000000000000000000, 0.000000000000000000, -200.0000000000000000 ) ) ;
#37429=DIRECTION ( 'NONE',  ( 0.000000000000000000, 0.000000000000000000, -1.000000000000000000 ) ) ;
#37587=CARTESIAN_POINT ( 'NONE',  ( 7.071067811865472841, -7.071067811865472841, -200.0000000000000000 ) ) ;
#37618=ORIENTED_EDGE ( 'NONE', *, *, #6976, .T. ) ;
#37668=VERTEX_POINT ( 'NONE', #4654 ) ;
#37722=DIRECTION ( 'NONE',  ( 0.000000000000000000, 0.08715574274765837404, -0.9961946980917455452 ) ) ;
#37885=FACE_OUTER_BOUND ( 'NONE', #2652, .T. ) ;
#37889=DIRECTION ( 'NONE',  ( 1.000000000000000000, 0.000000000000000000, 0.000000000000000000 ) ) ;
#37894=DIRECTION ( 'NONE',  ( 0.000000000000000000, 0.000000000000000000, 1.000000000000000000 ) ) ;
#37953=CARTESIAN_POINT ( 'NONE',  ( 42.00000000000001421, 5.327213576290987622E-15, -200.0000000000000000 ) ) ;
#38005=FACE_OUTER_BOUND ( 'NONE', #18886, .T. ) ;
#38069=EDGE_CURVE ( 'NONE', #23937, #38155, #29495, .T. ) ;
#38093=ORIENTED_EDGE ( 'NONE', *, *, #31491, .F. ) ;
#38099=SHAPE_REPRESENTATION_RELATIONSHIP ( 'NONE' , 'NONE' ,  #36293, #29436 ) ;
#38116=DIRECTION ( 'NONE',  ( -0.08682659386424779191, 0.08682659386424779191, 0.9924325091389669673 ) ) ;
#38155=VERTEX_POINT ( 'NONE', #1636 ) ;
#38306=AXIS2_PLACEMENT_3D ( 'NONE', #4650, #7679, #34016 ) ;
#38318=ORIENTED_EDGE ( 'NONE', *, *, #42273, .T. ) ;
#38350=EDGE_CURVE ( 'NONE', #12651, #37668, #8326, .T. ) ;
#38359=DIRECTION ( 'NONE',  ( -1.000000000000000000, 0.000000000000000000, 0.000000000000000000 ) ) ;
#38427=DIRECTION ( 'NONE',  ( 1.000000000000000000, 0.000000000000000000, 0.000000000000000000 ) ) ;
#38517=ORIENTED_EDGE ( 'NONE', *, *, #16442, .F. ) ;
#38534=CARTESIAN_POINT ( 'NONE',  ( -6.964452268037473637, 6.964452268037472749, -201.2186212422413689 ) ) ;
#38638=VERTEX_POINT ( 'NONE', #19713 ) ;
#38801=DIRECTION ( 'NONE',  ( -0.000000000000000000, -0.000000000000000000, -1.000000000000000000 ) ) ;
#38996=CARTESIAN_POINT ( 'NONE',  ( 5.000000000000002665, 20.00000000000000000, -235.0000000000000000 ) ) ;
#39088=EDGE_LOOP ( 'NONE', ( #26162, #16309 ) ) ;
#39105=CYLINDRICAL_SURFACE ( 'NONE', #41882, 5.000000000000002665 ) ;
#39209=ORIENTED_EDGE ( 'NONE', *, *, #20300, .F. ) ;
#39432=CARTESIAN_POINT ( 'NONE',  ( 7.071067811865472841, 7.071067811865472841, -200.0000000000000000 ) ) ;
#39478=CARTESIAN_POINT ( 'NONE',  ( -5.321294541346989426, 5.321294541346989426, -219.9999999999999716 ) ) ;
#39677=VECTOR ( 'NONE', #14777, 1000.000000000000000 ) ;
#39837=EDGE_CURVE ( 'NONE', #32599, #3542, #31477, .T. ) ;
#39839=ORIENTED_EDGE ( 'NONE', *, *, #18037, .F. ) ;
#39844=DIRECTION ( 'NONE',  ( 1.000000000000000000, 0.000000000000000000, 0.000000000000000000 ) ) ;
#39890=EDGE_CURVE ( 'NONE', #12005, #21356, #19554, .T. ) ;
#39924=LINE ( 'NONE', #674, #3136 ) ;
#39929=DIRECTION ( 'NONE',  ( 0.000000000000000000, 0.000000000000000000, -1.000000000000000000 ) ) ;
#39980=AXIS2_PLACEMENT_3D ( 'NONE', #19139, #19343, #38359 ) ;
#39986=LINE ( 'NONE', #10417, #31165 ) ;
#39998=AXIS2_PLACEMENT_3D ( 'NONE', #24743, #11112, #37889 ) ;
#40001=CARTESIAN_POINT ( 'NONE',  ( 0.000000000000000000, 0.000000000000000000, -200.0000000000000000 ) ) ;
#40129=CARTESIAN_POINT ( 'NONE',  ( -5.000000000000005329, -20.00000000000000000, -235.0000000000000000 ) ) ;
#40340=ORIENTED_EDGE ( 'NONE', *, *, #31655, .T. ) ;
#40617=AXIS2_PLACEMENT_3D ( 'NONE', #17551, #30752, #4626 ) ;
#40709=EDGE_CURVE ( 'NONE', #12005, #13682, #7576, .T. ) ;
#40939=CYLINDRICAL_SURFACE ( 'NONE', #19340, 5.000000000000002665 ) ;
#41048=CARTESIAN_POINT ( 'NONE',  ( -7.071067811865472841, -7.071067811865472841, -200.0000000000000000 ) ) ;
#41100=LINE ( 'NONE', #22550, #1100 ) ;
#41214=EDGE_CURVE ( 'NONE', #20412, #21356, #15836, .T. ) ;
#41304=CARTESIAN_POINT ( 'NONE',  ( 5.000000000000000000, -20.00000000000000000, -235.0000000000000000 ) ) ;
#41769=CONICAL_SURFACE ( 'NONE', #23894, 42.00000000000004974, 0.7853981633974495002 ) ;
#41882=AXIS2_PLACEMENT_3D ( 'NONE', #16205, #3290, #23138 ) ;
#41889=CARTESIAN_POINT ( 'NONE',  ( -42.00000000000004974, 5.327213576290989989E-15, -219.9999999999999716 ) ) ;
#41891=DIRECTION ( 'NONE',  ( -1.000000000000000000, 0.000000000000000000, 0.000000000000000000 ) ) ;
#41976=CARTESIAN_POINT ( 'NONE',  ( 0.000000000000000000, 0.000000000000000000, -217.0000000000000853 ) ) ;
#42021=CARTESIAN_POINT ( 'NONE',  ( 0.000000000000000000, 0.000000000000000000, -203.0000000000000000 ) ) ;
#42117=PLANE ( 'NONE',  #14158 ) ;
#42165=VECTOR ( 'NONE', #32479, 1000.000000000000000 ) ;
#42236=CARTESIAN_POINT ( 'NONE',  ( 45.00000000000000711, 5.510910596163090344E-15, -203.0000000000000000 ) ) ;
#42273=EDGE_CURVE ( 'NONE', #13682, #20412, #31480, .T. ) ;
#42288=ADVANCED_FACE ( 'NONE', ( #34291 ), #40939, .T. ) ;
#42330=ORIENTED_EDGE ( 'NONE', *, *, #20300, .T. ) ;
#42386=DIRECTION ( 'NONE',  ( 0.000000000000000000, 0.000000000000000000, -1.000000000000000000 ) ) ;
#42426=FACE_OUTER_BOUND ( 'NONE', #37129, .T. ) ;
#42479=VECTOR ( 'NONE', #24335, 1000.000000000000000 ) ;
#42482=VERTEX_POINT ( 'NONE', #2552 ) ;
#42657=AXIS2_PLACEMENT_3D ( 'NONE', #5647, #31984, #31557 ) ;
#42704=COLOUR_RGB('Light Blue', 0.66274510, 0.83137255, 0.94901961);
#42705=FILL_AREA_STYLE_COLOUR('',#42704);
#42706=FILL_AREA_STYLE('',(#42705));
#42707=SURFACE_STYLE_FILL_AREA(#42706);
#42708=SURFACE_SIDE_STYLE('',(#42707));
#42709=SURFACE_STYLE_USAGE(.BOTH.,#42708);
#42710=PRESENTATION_STYLE_ASSIGNMENT((#42709));
#42747=STYLED_ITEM('',(#42710),#1487);
#42748=MECHANICAL_DESIGN_GEOMETRIC_PRESENTATION_REPRESENTATION('',(#42747),#13832);
ENDSEC;
END-ISO-10303-21;
